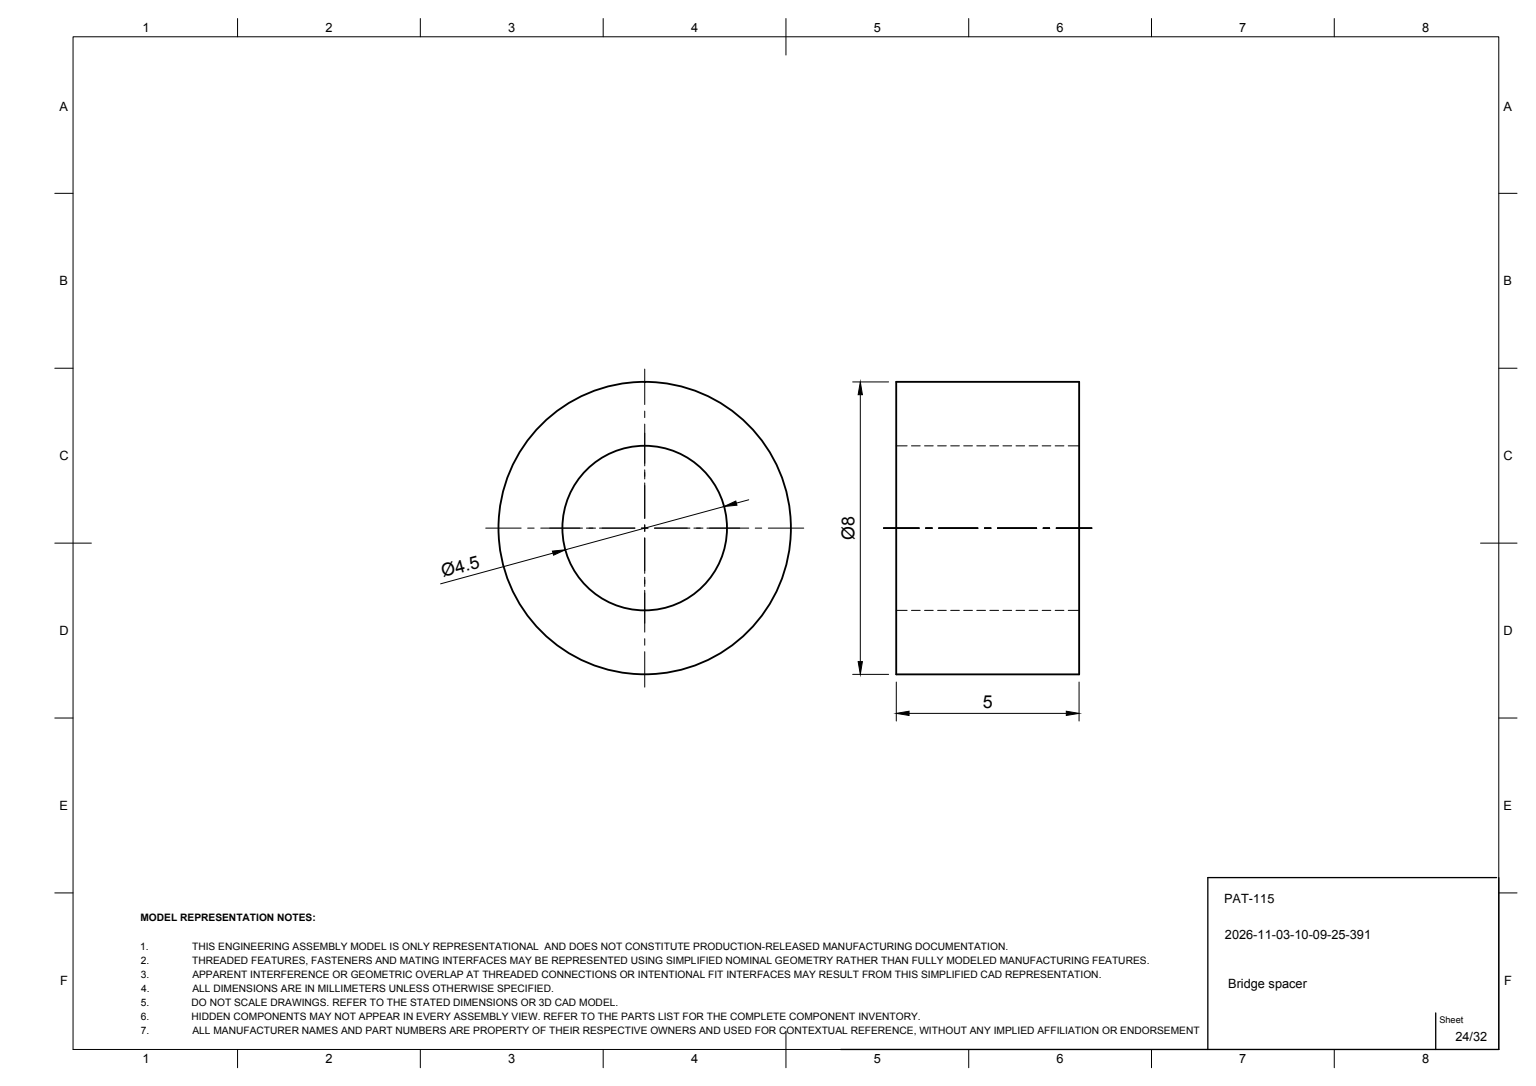
ISO-10303-21;
HEADER;
/* Generated by software containing ST-Developer
 * from STEP Tools, Inc. (www.steptools.com) 
 */

FILE_DESCRIPTION(
/* description */ ('Union bypass pipe loop'),
/* implementation_level */ '2;1');

FILE_NAME(
/* name */ 'Bridge spacer.step',
/* time_stamp */ '2026-10-27T21:00:29-07:00',
/* author */ (''),
/* organization */ (''),
/* preprocessor_version */ 'ST-DEVELOPER v20.2',
/* originating_system */ 'Autodesk Translation Framework v15.17.0.0',
/* authorisation */ '');

FILE_SCHEMA (('AUTOMOTIVE_DESIGN { 1 0 10303 214 3 1 1 }'));
ENDSEC;

DATA;
#10=MECHANICAL_DESIGN_GEOMETRIC_PRESENTATION_REPRESENTATION('',(#456),#10095);
#392=SHAPE_REPRESENTATION_RELATIONSHIP('SRR','None',#10261,#424);
#424=ADVANCED_BREP_SHAPE_REPRESENTATION('',(#487),#10073);
#456=STYLED_ITEM('',(#10493),#487);
#487=MANIFOLD_SOLID_BREP('Body1',#5528);
#574=FACE_BOUND('',#1358,.T.);
#575=FACE_BOUND('',#1360,.T.);
#706=PLANE('',#6154);
#707=PLANE('',#6155);
#960=FACE_OUTER_BOUND('',#1355,.T.);
#961=FACE_OUTER_BOUND('',#1356,.T.);
#962=FACE_OUTER_BOUND('',#1357,.T.);
#963=FACE_OUTER_BOUND('',#1359,.T.);
#1355=EDGE_LOOP('',(#4258,#4259,#4260,#4261));
#1356=EDGE_LOOP('',(#4262,#4263,#4264,#4265));
#1357=EDGE_LOOP('',(#4266));
#1358=EDGE_LOOP('',(#4267));
#1359=EDGE_LOOP('',(#4268));
#1360=EDGE_LOOP('',(#4269));
#1768=LINE('',#9023,#2144);
#1769=LINE('',#9029,#2145);
#2144=VECTOR('',#7254,0.225);
#2145=VECTOR('',#7261,0.4);
#2478=CIRCLE('',#6149,0.225);
#2479=CIRCLE('',#6150,0.225);
#2480=CIRCLE('',#6152,0.4);
#2481=CIRCLE('',#6153,0.4);
#2802=VERTEX_POINT('',#9020);
#2803=VERTEX_POINT('',#9022);
#2804=VERTEX_POINT('',#9026);
#2805=VERTEX_POINT('',#9028);
#3327=EDGE_CURVE('',#2802,#2802,#2478,.T.);
#3328=EDGE_CURVE('',#2802,#2803,#1768,.T.);
#3329=EDGE_CURVE('',#2803,#2803,#2479,.T.);
#3330=EDGE_CURVE('',#2804,#2804,#2480,.T.);
#3331=EDGE_CURVE('',#2804,#2805,#1769,.T.);
#3332=EDGE_CURVE('',#2805,#2805,#2481,.T.);
#4258=ORIENTED_EDGE('',*,*,#3327,.F.);
#4259=ORIENTED_EDGE('',*,*,#3328,.T.);
#4260=ORIENTED_EDGE('',*,*,#3329,.T.);
#4261=ORIENTED_EDGE('',*,*,#3328,.F.);
#4262=ORIENTED_EDGE('',*,*,#3330,.F.);
#4263=ORIENTED_EDGE('',*,*,#3331,.T.);
#4264=ORIENTED_EDGE('',*,*,#3332,.T.);
#4265=ORIENTED_EDGE('',*,*,#3331,.F.);
#4266=ORIENTED_EDGE('',*,*,#3330,.T.);
#4267=ORIENTED_EDGE('',*,*,#3327,.T.);
#4268=ORIENTED_EDGE('',*,*,#3332,.F.);
#4269=ORIENTED_EDGE('',*,*,#3329,.F.);
#5124=CYLINDRICAL_SURFACE('',#6148,0.225);
#5125=CYLINDRICAL_SURFACE('',#6151,0.4);
#5309=ADVANCED_FACE('',(#960),#5124,.F.);
#5310=ADVANCED_FACE('',(#961),#5125,.T.);
#5311=ADVANCED_FACE('',(#962,#574),#706,.T.);
#5312=ADVANCED_FACE('',(#963,#575),#707,.F.);
#5528=CLOSED_SHELL('',(#5309,#5310,#5311,#5312));
#6147=AXIS2_PLACEMENT_3D('',#9018,#7248,#7249);
#6148=AXIS2_PLACEMENT_3D('',#9019,#7250,#7251);
#6149=AXIS2_PLACEMENT_3D('',#9021,#7252,#7253);
#6150=AXIS2_PLACEMENT_3D('',#9024,#7255,#7256);
#6151=AXIS2_PLACEMENT_3D('',#9025,#7257,#7258);
#6152=AXIS2_PLACEMENT_3D('',#9027,#7259,#7260);
#6153=AXIS2_PLACEMENT_3D('',#9030,#7262,#7263);
#6154=AXIS2_PLACEMENT_3D('',#9031,#7264,#7265);
#6155=AXIS2_PLACEMENT_3D('',#9032,#7266,#7267);
#7248=DIRECTION('axis',(0.,0.,1.));
#7249=DIRECTION('refdir',(1.,0.,0.));
#7250=DIRECTION('center_axis',(0.,0.,1.));
#7251=DIRECTION('ref_axis',(1.,0.,0.));
#7252=DIRECTION('center_axis',(0.,0.,-1.));
#7253=DIRECTION('ref_axis',(1.,0.,0.));
#7254=DIRECTION('',(0.,0.,-1.));
#7255=DIRECTION('center_axis',(0.,0.,-1.));
#7256=DIRECTION('ref_axis',(1.,0.,0.));
#7257=DIRECTION('center_axis',(0.,0.,1.));
#7258=DIRECTION('ref_axis',(1.,0.,0.));
#7259=DIRECTION('center_axis',(0.,0.,1.));
#7260=DIRECTION('ref_axis',(1.,0.,0.));
#7261=DIRECTION('',(0.,0.,-1.));
#7262=DIRECTION('center_axis',(0.,0.,1.));
#7263=DIRECTION('ref_axis',(1.,0.,0.));
#7264=DIRECTION('center_axis',(0.,0.,1.));
#7265=DIRECTION('ref_axis',(1.,0.,0.));
#7266=DIRECTION('center_axis',(0.,0.,1.));
#7267=DIRECTION('ref_axis',(1.,0.,0.));
#9018=CARTESIAN_POINT('',(0.,0.,0.));
#9019=CARTESIAN_POINT('Origin',(-1.3,-1.,7.5));
#9020=CARTESIAN_POINT('',(-1.525,-1.,8.));
#9021=CARTESIAN_POINT('Origin',(-1.3,-1.,8.));
#9022=CARTESIAN_POINT('',(-1.525,-1.,7.5));
#9023=CARTESIAN_POINT('',(-1.525,-1.,7.5));
#9024=CARTESIAN_POINT('Origin',(-1.3,-1.,7.5));
#9025=CARTESIAN_POINT('Origin',(-1.3,-1.,7.5));
#9026=CARTESIAN_POINT('',(-1.7,-1.,8.));
#9027=CARTESIAN_POINT('Origin',(-1.3,-1.,8.));
#9028=CARTESIAN_POINT('',(-1.7,-1.,7.5));
#9029=CARTESIAN_POINT('',(-1.7,-1.,7.5));
#9030=CARTESIAN_POINT('Origin',(-1.3,-1.,7.5));
#9031=CARTESIAN_POINT('Origin',(-1.3,-1.,8.));
#9032=CARTESIAN_POINT('Origin',(-1.3,-1.,7.5));
#10036=UNCERTAINTY_MEASURE_WITH_UNIT(LENGTH_MEASURE(0.001),#10096,
'DISTANCE_ACCURACY_VALUE',
'Maximum model space distance between geometric entities at asserted c
onnectivities');
#10058=UNCERTAINTY_MEASURE_WITH_UNIT(LENGTH_MEASURE(0.001),#10096,
'DISTANCE_ACCURACY_VALUE',
'Maximum model space distance between geometric entities at asserted c
onnectivities');
#10073=(
GEOMETRIC_REPRESENTATION_CONTEXT(3)
GLOBAL_UNCERTAINTY_ASSIGNED_CONTEXT((#10036))
GLOBAL_UNIT_ASSIGNED_CONTEXT((#10096,#10098,#10099))
REPRESENTATION_CONTEXT('','3D')
);
#10095=(
GEOMETRIC_REPRESENTATION_CONTEXT(3)
GLOBAL_UNCERTAINTY_ASSIGNED_CONTEXT((#10058))
GLOBAL_UNIT_ASSIGNED_CONTEXT((#10096,#10098,#10099))
REPRESENTATION_CONTEXT('','3D')
);
#10096=(
LENGTH_UNIT()
NAMED_UNIT(*)
SI_UNIT(.CENTI.,.METRE.)
);
#10098=(
NAMED_UNIT(*)
PLANE_ANGLE_UNIT()
SI_UNIT($,.RADIAN.)
);
#10099=(
NAMED_UNIT(*)
SI_UNIT($,.STERADIAN.)
SOLID_ANGLE_UNIT()
);
#10114=SHAPE_DEFINITION_REPRESENTATION(#10150,#10261);
#10150=PRODUCT_DEFINITION_SHAPE('',$,#10298);
#10261=SHAPE_REPRESENTATION('',(#6147),#10073);
#10283=PRODUCT_DEFINITION_CONTEXT('part definition',#10393,'design');
#10298=PRODUCT_DEFINITION('Bridge spacer','Bridge spacer',#10334,#10283);
#10334=PRODUCT_DEFINITION_FORMATION('',$,#10409);
#10393=APPLICATION_CONTEXT(
'Core Data for Automotive Mechanical Design Process');
#10394=PRODUCT_CONTEXT('part definition',#10393,'mechanical');
#10409=PRODUCT('Bridge spacer','Bridge spacer','Bridge spacer',(#10394));
#10487=COLOUR_RGB('Sky Blue',0.24,0.69,0.87);
#10488=FILL_AREA_STYLE_COLOUR('',#10487);
#10489=FILL_AREA_STYLE('',(#10488));
#10490=SURFACE_STYLE_FILL_AREA(#10489);
#10491=SURFACE_SIDE_STYLE('',(#10490));
#10492=SURFACE_STYLE_USAGE(.BOTH.,#10491);
#10493=PRESENTATION_STYLE_ASSIGNMENT((#10492));
ENDSEC;
END-ISO-10303-21;
